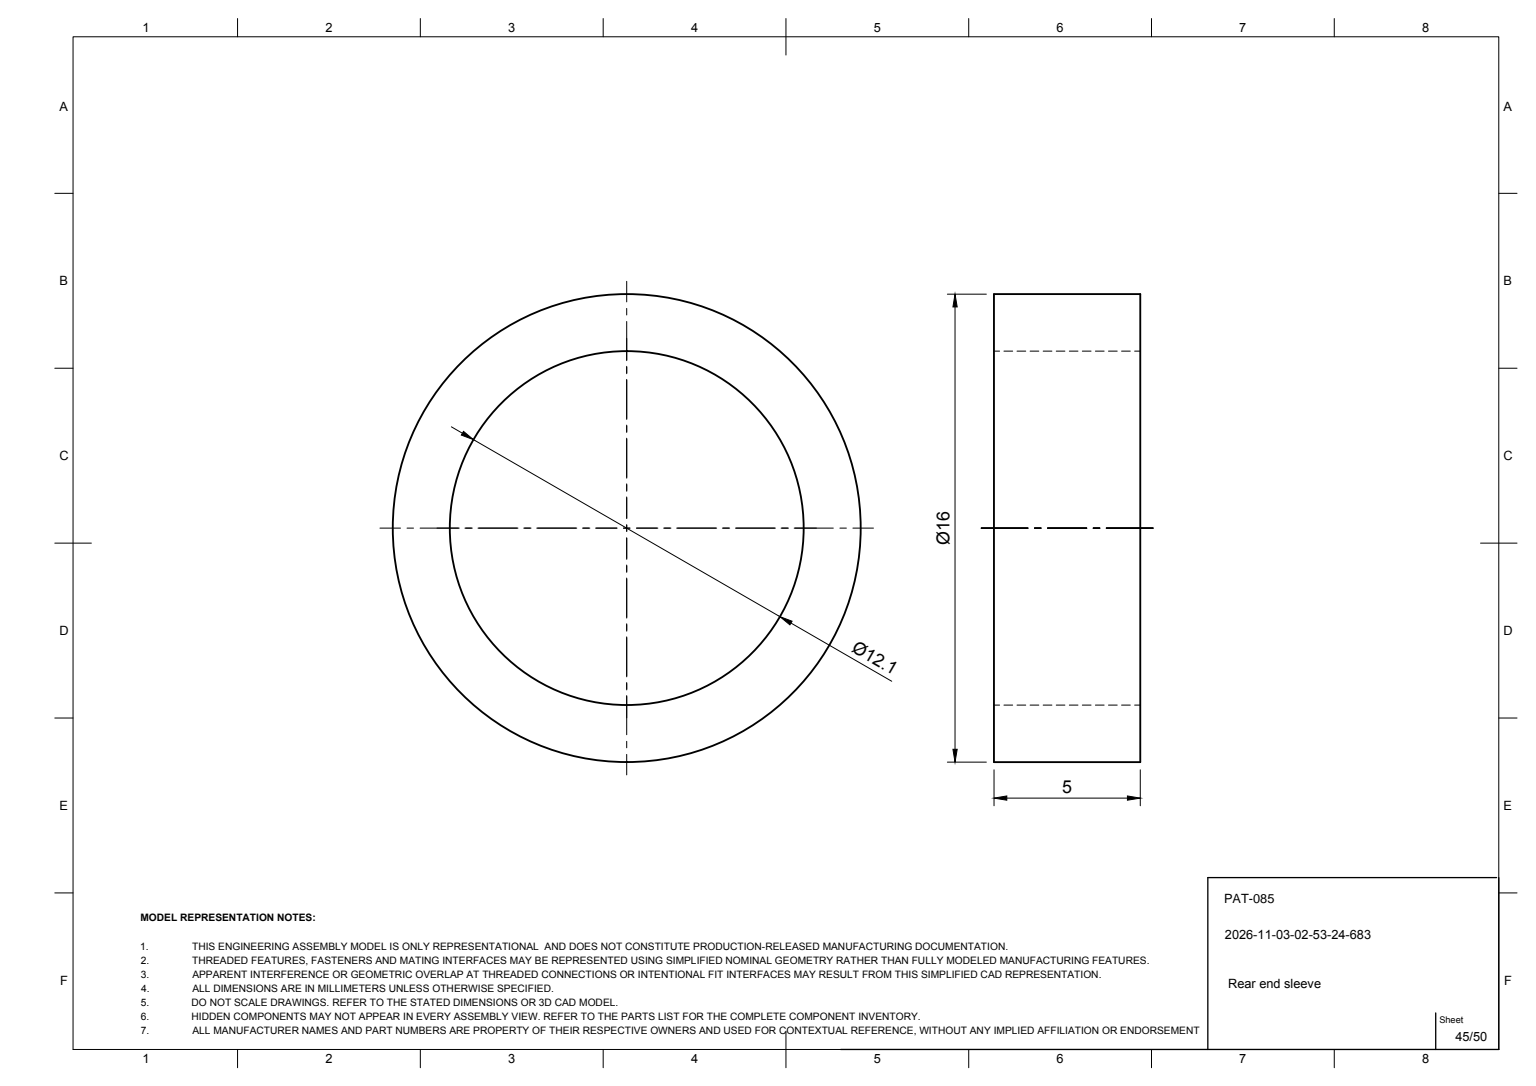
ISO-10303-21;
HEADER;
/* Generated by software containing ST-Developer
 * from STEP Tools, Inc. (www.steptools.com) 
 */

FILE_DESCRIPTION(
/* description */ ('Rack and pinion manual slide'),
/* implementation_level */ '2;1');

FILE_NAME(
/* name */ 'Rear end sleeve.step',
/* time_stamp */ '2026-10-28T03:22:49-07:00',
/* author */ (''),
/* organization */ (''),
/* preprocessor_version */ 'ST-DEVELOPER v20.2',
/* originating_system */ 'Autodesk Translation Framework v15.17.0.0',
/* authorisation */ '');

FILE_SCHEMA (('AUTOMOTIVE_DESIGN { 1 0 10303 214 3 1 1 }'));
ENDSEC;

DATA;
#10=MECHANICAL_DESIGN_GEOMETRIC_PRESENTATION_REPRESENTATION('',(#776),#34851);
#677=SHAPE_REPRESENTATION_RELATIONSHIP('SRR','None',#35116,#723);
#723=ADVANCED_BREP_SHAPE_REPRESENTATION('',(#826),#34841);
#776=STYLED_ITEM('',(#35404),#826);
#826=MANIFOLD_SOLID_BREP('Body1',#13799);
#1026=FACE_BOUND('',#3048,.T.);
#1027=FACE_BOUND('',#3050,.T.);
#1460=PLANE('',#15287);
#1461=PLANE('',#15288);
#2113=FACE_OUTER_BOUND('',#3045,.T.);
#2114=FACE_OUTER_BOUND('',#3046,.T.);
#2115=FACE_OUTER_BOUND('',#3047,.T.);
#2116=FACE_OUTER_BOUND('',#3049,.T.);
#3045=EDGE_LOOP('',(#12050,#12051,#12052,#12053));
#3046=EDGE_LOOP('',(#12054,#12055,#12056,#12057));
#3047=EDGE_LOOP('',(#12058));
#3048=EDGE_LOOP('',(#12059));
#3049=EDGE_LOOP('',(#12060));
#3050=EDGE_LOOP('',(#12061));
#4284=LINE('',#22736,#5575);
#4285=LINE('',#22742,#5576);
#5575=VECTOR('',#18592,0.605);
#5576=VECTOR('',#18599,0.800000000000001);
#6138=CIRCLE('',#15282,0.605);
#6139=CIRCLE('',#15283,0.605);
#6140=CIRCLE('',#15285,0.800000000000001);
#6141=CIRCLE('',#15286,0.800000000000001);
#7167=VERTEX_POINT('',#22733);
#7168=VERTEX_POINT('',#22735);
#7169=VERTEX_POINT('',#22739);
#7170=VERTEX_POINT('',#22741);
#8837=EDGE_CURVE('',#7167,#7167,#6138,.T.);
#8838=EDGE_CURVE('',#7167,#7168,#4284,.T.);
#8839=EDGE_CURVE('',#7168,#7168,#6139,.T.);
#8840=EDGE_CURVE('',#7169,#7169,#6140,.T.);
#8841=EDGE_CURVE('',#7169,#7170,#4285,.T.);
#8842=EDGE_CURVE('',#7170,#7170,#6141,.T.);
#12050=ORIENTED_EDGE('',*,*,#8837,.F.);
#12051=ORIENTED_EDGE('',*,*,#8838,.T.);
#12052=ORIENTED_EDGE('',*,*,#8839,.T.);
#12053=ORIENTED_EDGE('',*,*,#8838,.F.);
#12054=ORIENTED_EDGE('',*,*,#8840,.F.);
#12055=ORIENTED_EDGE('',*,*,#8841,.T.);
#12056=ORIENTED_EDGE('',*,*,#8842,.T.);
#12057=ORIENTED_EDGE('',*,*,#8841,.F.);
#12058=ORIENTED_EDGE('',*,*,#8840,.T.);
#12059=ORIENTED_EDGE('',*,*,#8837,.T.);
#12060=ORIENTED_EDGE('',*,*,#8842,.F.);
#12061=ORIENTED_EDGE('',*,*,#8839,.F.);
#12975=CYLINDRICAL_SURFACE('',#15281,0.605);
#12976=CYLINDRICAL_SURFACE('',#15284,0.800000000000001);
#13591=ADVANCED_FACE('',(#2113),#12975,.F.);
#13592=ADVANCED_FACE('',(#2114),#12976,.T.);
#13593=ADVANCED_FACE('',(#2115,#1026),#1460,.T.);
#13594=ADVANCED_FACE('',(#2116,#1027),#1461,.F.);
#13799=CLOSED_SHELL('',(#13591,#13592,#13593,#13594));
#15280=AXIS2_PLACEMENT_3D('',#22731,#18586,#18587);
#15281=AXIS2_PLACEMENT_3D('',#22732,#18588,#18589);
#15282=AXIS2_PLACEMENT_3D('',#22734,#18590,#18591);
#15283=AXIS2_PLACEMENT_3D('',#22737,#18593,#18594);
#15284=AXIS2_PLACEMENT_3D('',#22738,#18595,#18596);
#15285=AXIS2_PLACEMENT_3D('',#22740,#18597,#18598);
#15286=AXIS2_PLACEMENT_3D('',#22743,#18600,#18601);
#15287=AXIS2_PLACEMENT_3D('',#22744,#18602,#18603);
#15288=AXIS2_PLACEMENT_3D('',#22745,#18604,#18605);
#18586=DIRECTION('axis',(0.,0.,1.));
#18587=DIRECTION('refdir',(1.,0.,0.));
#18588=DIRECTION('center_axis',(0.,1.,0.));
#18589=DIRECTION('ref_axis',(1.,0.,0.));
#18590=DIRECTION('center_axis',(0.,-1.,0.));
#18591=DIRECTION('ref_axis',(1.,0.,0.));
#18592=DIRECTION('',(0.,-1.,0.));
#18593=DIRECTION('center_axis',(0.,-1.,0.));
#18594=DIRECTION('ref_axis',(1.,0.,0.));
#18595=DIRECTION('center_axis',(0.,1.,0.));
#18596=DIRECTION('ref_axis',(1.,0.,0.));
#18597=DIRECTION('center_axis',(0.,1.,0.));
#18598=DIRECTION('ref_axis',(1.,0.,0.));
#18599=DIRECTION('',(0.,-1.,0.));
#18600=DIRECTION('center_axis',(0.,1.,0.));
#18601=DIRECTION('ref_axis',(1.,0.,0.));
#18602=DIRECTION('center_axis',(0.,1.,0.));
#18603=DIRECTION('ref_axis',(1.,0.,0.));
#18604=DIRECTION('center_axis',(0.,1.,0.));
#18605=DIRECTION('ref_axis',(1.,0.,0.));
#22731=CARTESIAN_POINT('',(0.,0.,0.));
#22732=CARTESIAN_POINT('Origin',(11.,-6.5,10.25));
#22733=CARTESIAN_POINT('',(10.395,-6.,10.25));
#22734=CARTESIAN_POINT('Origin',(11.,-6.,10.25));
#22735=CARTESIAN_POINT('',(10.395,-6.5,10.25));
#22736=CARTESIAN_POINT('',(10.395,-6.5,10.25));
#22737=CARTESIAN_POINT('Origin',(11.,-6.5,10.25));
#22738=CARTESIAN_POINT('Origin',(11.,-6.5,10.25));
#22739=CARTESIAN_POINT('',(10.2,-6.,10.25));
#22740=CARTESIAN_POINT('Origin',(11.,-6.,10.25));
#22741=CARTESIAN_POINT('',(10.2,-6.5,10.25));
#22742=CARTESIAN_POINT('',(10.2,-6.5,10.25));
#22743=CARTESIAN_POINT('Origin',(11.,-6.5,10.25));
#22744=CARTESIAN_POINT('Origin',(11.,-6.,10.25));
#22745=CARTESIAN_POINT('Origin',(11.,-6.5,10.25));
#34787=UNCERTAINTY_MEASURE_WITH_UNIT(LENGTH_MEASURE(0.001),#34852,
'DISTANCE_ACCURACY_VALUE',
'Maximum model space distance between geometric entities at asserted c
onnectivities');
#34797=UNCERTAINTY_MEASURE_WITH_UNIT(LENGTH_MEASURE(0.001),#34852,
'DISTANCE_ACCURACY_VALUE',
'Maximum model space distance between geometric entities at asserted c
onnectivities');
#34841=(
GEOMETRIC_REPRESENTATION_CONTEXT(3)
GLOBAL_UNCERTAINTY_ASSIGNED_CONTEXT((#34787))
GLOBAL_UNIT_ASSIGNED_CONTEXT((#34852,#34854,#34855))
REPRESENTATION_CONTEXT('','3D')
);
#34851=(
GEOMETRIC_REPRESENTATION_CONTEXT(3)
GLOBAL_UNCERTAINTY_ASSIGNED_CONTEXT((#34797))
GLOBAL_UNIT_ASSIGNED_CONTEXT((#34852,#34854,#34855))
REPRESENTATION_CONTEXT('','3D')
);
#34852=(
LENGTH_UNIT()
NAMED_UNIT(*)
SI_UNIT(.CENTI.,.METRE.)
);
#34854=(
NAMED_UNIT(*)
PLANE_ANGLE_UNIT()
SI_UNIT($,.RADIAN.)
);
#34855=(
NAMED_UNIT(*)
SI_UNIT($,.STERADIAN.)
SOLID_ANGLE_UNIT()
);
#34899=SHAPE_DEFINITION_REPRESENTATION(#34960,#35116);
#34960=PRODUCT_DEFINITION_SHAPE('',$,#35170);
#35116=SHAPE_REPRESENTATION('',(#15280),#34841);
#35126=PRODUCT_DEFINITION_CONTEXT('part definition',#35287,'design');
#35170=PRODUCT_DEFINITION('Rear end sleeve','Rear end sleeve',#35223,#35126);
#35223=PRODUCT_DEFINITION_FORMATION('',$,#35332);
#35287=APPLICATION_CONTEXT(
'Core Data for Automotive Mechanical Design Process');
#35288=PRODUCT_CONTEXT('part definition',#35287,'mechanical');
#35332=PRODUCT('Rear end sleeve','Rear end sleeve','Rear end sleeve',(#35288));
#35398=COLOUR_RGB('Sky Blue',0.24,0.69,0.87);
#35399=FILL_AREA_STYLE_COLOUR('',#35398);
#35400=FILL_AREA_STYLE('',(#35399));
#35401=SURFACE_STYLE_FILL_AREA(#35400);
#35402=SURFACE_SIDE_STYLE('',(#35401));
#35403=SURFACE_STYLE_USAGE(.BOTH.,#35402);
#35404=PRESENTATION_STYLE_ASSIGNMENT((#35403));
ENDSEC;
END-ISO-10303-21;
